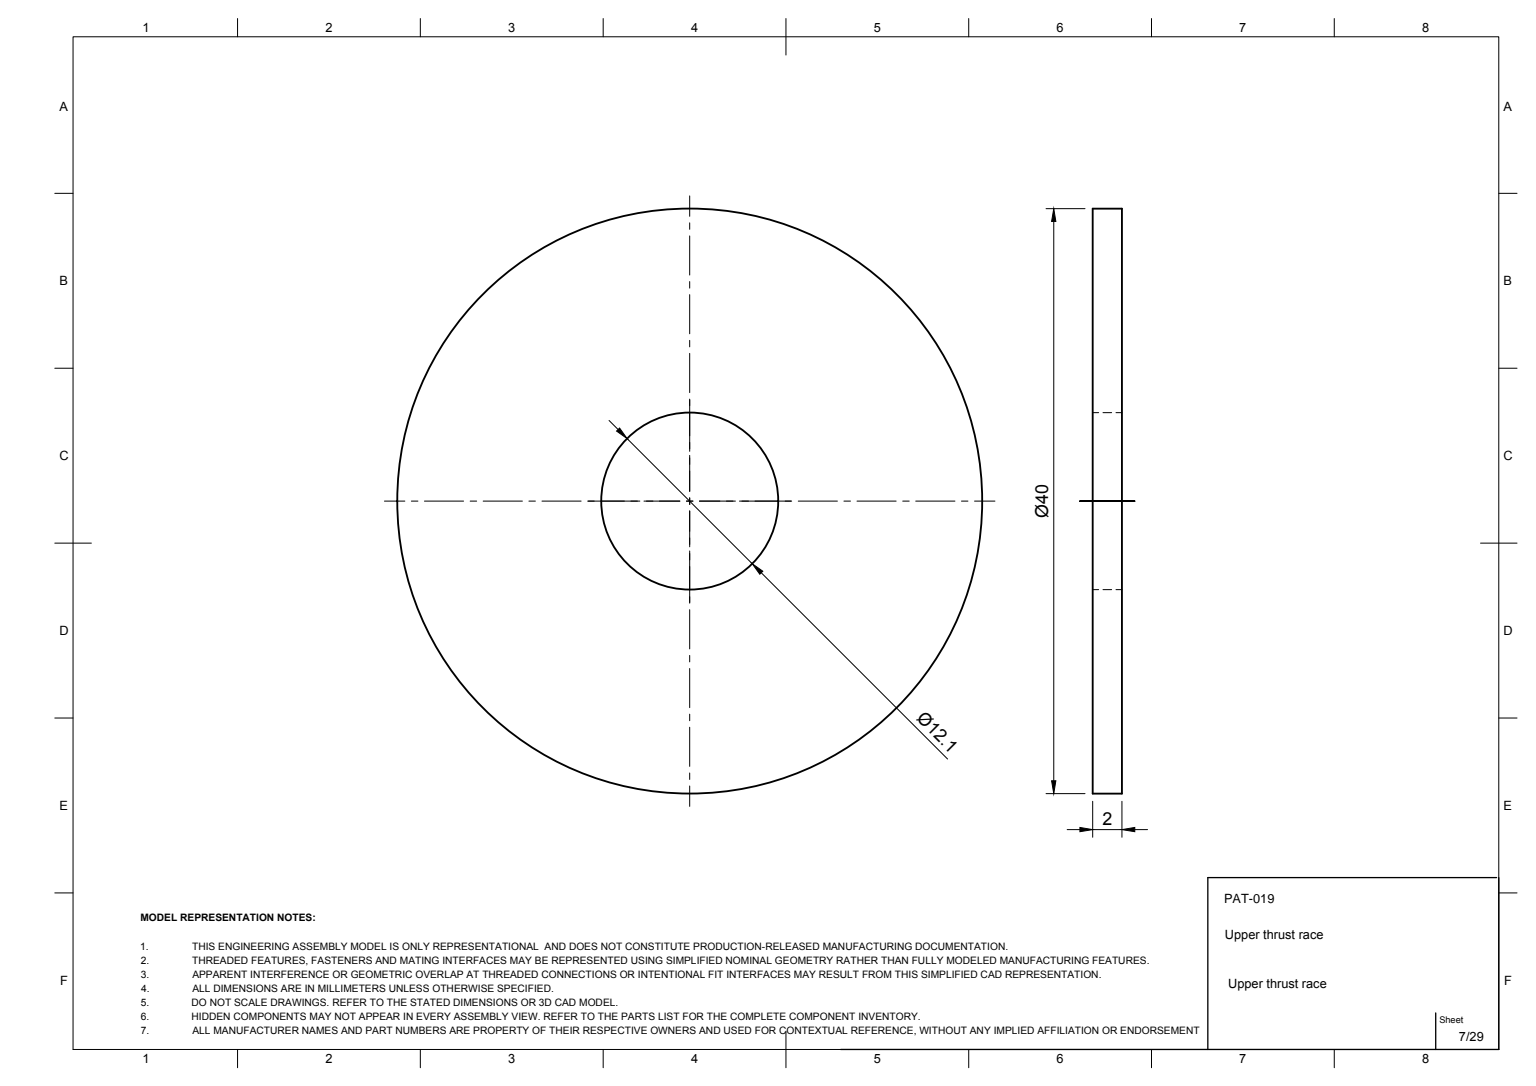
ISO-10303-21;
HEADER;
/* Generated by software containing ST-Developer
 * from STEP Tools, Inc. (www.steptools.com) 
 */

FILE_DESCRIPTION(
/* description */ ('Caster wheel assembly'),
/* implementation_level */ '2;1');

FILE_NAME(
/* name */ 'Upper thrust race.step',
/* time_stamp */ '2026-10-28T03:23:56-07:00',
/* author */ (''),
/* organization */ (''),
/* preprocessor_version */ 'ST-DEVELOPER v20.2',
/* originating_system */ 'Autodesk Translation Framework v15.17.0.0',
/* authorisation */ '');

FILE_SCHEMA (('AUTOMOTIVE_DESIGN { 1 0 10303 214 3 1 1 }'));
ENDSEC;

DATA;
#10=MECHANICAL_DESIGN_GEOMETRIC_PRESENTATION_REPRESENTATION('',(#224),#5385);
#180=SHAPE_REPRESENTATION_RELATIONSHIP('SRR','None',#5475,#202);
#202=ADVANCED_BREP_SHAPE_REPRESENTATION('',(#254),#5362);
#224=STYLED_ITEM('',(#5658),#254);
#254=MANIFOLD_SOLID_BREP('Body1',#2651);
#293=FACE_BOUND('',#622,.T.);
#294=FACE_BOUND('',#624,.T.);
#343=PLANE('',#2968);
#344=PLANE('',#2969);
#439=FACE_OUTER_BOUND('',#619,.T.);
#440=FACE_OUTER_BOUND('',#620,.T.);
#441=FACE_OUTER_BOUND('',#621,.T.);
#442=FACE_OUTER_BOUND('',#623,.T.);
#619=EDGE_LOOP('',(#1854,#1855,#1856,#1857));
#620=EDGE_LOOP('',(#1858,#1859,#1860,#1861));
#621=EDGE_LOOP('',(#1862));
#622=EDGE_LOOP('',(#1863));
#623=EDGE_LOOP('',(#1864));
#624=EDGE_LOOP('',(#1865));
#829=LINE('',#4287,#963);
#830=LINE('',#4293,#964);
#963=VECTOR('',#3406,0.605);
#964=VECTOR('',#3413,2.);
#1093=CIRCLE('',#2963,0.605);
#1094=CIRCLE('',#2964,0.605);
#1095=CIRCLE('',#2966,2.);
#1096=CIRCLE('',#2967,2.);
#1260=VERTEX_POINT('',#4284);
#1261=VERTEX_POINT('',#4286);
#1262=VERTEX_POINT('',#4290);
#1263=VERTEX_POINT('',#4292);
#1495=EDGE_CURVE('',#1260,#1260,#1093,.T.);
#1496=EDGE_CURVE('',#1260,#1261,#829,.T.);
#1497=EDGE_CURVE('',#1261,#1261,#1094,.T.);
#1498=EDGE_CURVE('',#1262,#1262,#1095,.T.);
#1499=EDGE_CURVE('',#1262,#1263,#830,.T.);
#1500=EDGE_CURVE('',#1263,#1263,#1096,.T.);
#1854=ORIENTED_EDGE('',*,*,#1495,.F.);
#1855=ORIENTED_EDGE('',*,*,#1496,.T.);
#1856=ORIENTED_EDGE('',*,*,#1497,.T.);
#1857=ORIENTED_EDGE('',*,*,#1496,.F.);
#1858=ORIENTED_EDGE('',*,*,#1498,.F.);
#1859=ORIENTED_EDGE('',*,*,#1499,.T.);
#1860=ORIENTED_EDGE('',*,*,#1500,.T.);
#1861=ORIENTED_EDGE('',*,*,#1499,.F.);
#1862=ORIENTED_EDGE('',*,*,#1498,.T.);
#1863=ORIENTED_EDGE('',*,*,#1495,.T.);
#1864=ORIENTED_EDGE('',*,*,#1500,.F.);
#1865=ORIENTED_EDGE('',*,*,#1497,.F.);
#2436=CYLINDRICAL_SURFACE('',#2962,0.605);
#2437=CYLINDRICAL_SURFACE('',#2965,2.);
#2499=ADVANCED_FACE('',(#439),#2436,.F.);
#2500=ADVANCED_FACE('',(#440),#2437,.T.);
#2501=ADVANCED_FACE('',(#441,#293),#343,.T.);
#2502=ADVANCED_FACE('',(#442,#294),#344,.F.);
#2651=CLOSED_SHELL('',(#2499,#2500,#2501,#2502));
#2961=AXIS2_PLACEMENT_3D('',#4282,#3400,#3401);
#2962=AXIS2_PLACEMENT_3D('',#4283,#3402,#3403);
#2963=AXIS2_PLACEMENT_3D('',#4285,#3404,#3405);
#2964=AXIS2_PLACEMENT_3D('',#4288,#3407,#3408);
#2965=AXIS2_PLACEMENT_3D('',#4289,#3409,#3410);
#2966=AXIS2_PLACEMENT_3D('',#4291,#3411,#3412);
#2967=AXIS2_PLACEMENT_3D('',#4294,#3414,#3415);
#2968=AXIS2_PLACEMENT_3D('',#4295,#3416,#3417);
#2969=AXIS2_PLACEMENT_3D('',#4296,#3418,#3419);
#3400=DIRECTION('axis',(0.,0.,1.));
#3401=DIRECTION('refdir',(1.,0.,0.));
#3402=DIRECTION('center_axis',(0.,0.,1.));
#3403=DIRECTION('ref_axis',(1.,0.,0.));
#3404=DIRECTION('center_axis',(0.,0.,-1.));
#3405=DIRECTION('ref_axis',(1.,0.,0.));
#3406=DIRECTION('',(0.,0.,-1.));
#3407=DIRECTION('center_axis',(0.,0.,-1.));
#3408=DIRECTION('ref_axis',(1.,0.,0.));
#3409=DIRECTION('center_axis',(0.,0.,1.));
#3410=DIRECTION('ref_axis',(1.,0.,0.));
#3411=DIRECTION('center_axis',(0.,0.,1.));
#3412=DIRECTION('ref_axis',(1.,0.,0.));
#3413=DIRECTION('',(0.,0.,-1.));
#3414=DIRECTION('center_axis',(0.,0.,1.));
#3415=DIRECTION('ref_axis',(1.,0.,0.));
#3416=DIRECTION('center_axis',(0.,0.,1.));
#3417=DIRECTION('ref_axis',(1.,0.,0.));
#3418=DIRECTION('center_axis',(0.,0.,1.));
#3419=DIRECTION('ref_axis',(1.,0.,0.));
#4282=CARTESIAN_POINT('',(0.,0.,0.));
#4283=CARTESIAN_POINT('Origin',(-2.,0.,9.5));
#4284=CARTESIAN_POINT('',(-2.605,-7.40911313484149E-17,9.7));
#4285=CARTESIAN_POINT('Origin',(-2.,0.,9.7));
#4286=CARTESIAN_POINT('',(-2.605,-7.40911313484149E-17,9.5));
#4287=CARTESIAN_POINT('',(-2.605,-7.40911313484149E-17,9.5));
#4288=CARTESIAN_POINT('Origin',(-2.,0.,9.5));
#4289=CARTESIAN_POINT('Origin',(-2.,0.,9.5));
#4290=CARTESIAN_POINT('',(-4.,-2.44929359829471E-16,9.7));
#4291=CARTESIAN_POINT('Origin',(-2.,0.,9.7));
#4292=CARTESIAN_POINT('',(-4.,-2.44929359829471E-16,9.5));
#4293=CARTESIAN_POINT('',(-4.,-2.44929359829471E-16,9.5));
#4294=CARTESIAN_POINT('Origin',(-2.,0.,9.5));
#4295=CARTESIAN_POINT('Origin',(-2.,0.,9.7));
#4296=CARTESIAN_POINT('Origin',(-2.,0.,9.5));
#5334=UNCERTAINTY_MEASURE_WITH_UNIT(LENGTH_MEASURE(0.001),#5386,
'DISTANCE_ACCURACY_VALUE',
'Maximum model space distance between geometric entities at asserted c
onnectivities');
#5357=UNCERTAINTY_MEASURE_WITH_UNIT(LENGTH_MEASURE(0.001),#5386,
'DISTANCE_ACCURACY_VALUE',
'Maximum model space distance between geometric entities at asserted c
onnectivities');
#5362=(
GEOMETRIC_REPRESENTATION_CONTEXT(3)
GLOBAL_UNCERTAINTY_ASSIGNED_CONTEXT((#5334))
GLOBAL_UNIT_ASSIGNED_CONTEXT((#5386,#5388,#5389))
REPRESENTATION_CONTEXT('','3D')
);
#5385=(
GEOMETRIC_REPRESENTATION_CONTEXT(3)
GLOBAL_UNCERTAINTY_ASSIGNED_CONTEXT((#5357))
GLOBAL_UNIT_ASSIGNED_CONTEXT((#5386,#5388,#5389))
REPRESENTATION_CONTEXT('','3D')
);
#5386=(
LENGTH_UNIT()
NAMED_UNIT(*)
SI_UNIT(.CENTI.,.METRE.)
);
#5388=(
NAMED_UNIT(*)
PLANE_ANGLE_UNIT()
SI_UNIT($,.RADIAN.)
);
#5389=(
NAMED_UNIT(*)
SI_UNIT($,.STERADIAN.)
SOLID_ANGLE_UNIT()
);
#5394=SHAPE_DEFINITION_REPRESENTATION(#5421,#5475);
#5421=PRODUCT_DEFINITION_SHAPE('',$,#5503);
#5475=SHAPE_REPRESENTATION('',(#2961),#5362);
#5498=PRODUCT_DEFINITION_CONTEXT('part definition',#5581,'design');
#5503=PRODUCT_DEFINITION('Upper thrust race','Upper thrust race',#5530,
#5498);
#5530=PRODUCT_DEFINITION_FORMATION('',$,#5587);
#5581=APPLICATION_CONTEXT(
'Core Data for Automotive Mechanical Design Process');
#5582=PRODUCT_CONTEXT('part definition',#5581,'mechanical');
#5587=PRODUCT('Upper thrust race','Upper thrust race',
'Upper thrust race',(#5582));
#5652=COLOUR_RGB('Light Blue',0.38,0.62,0.78);
#5653=FILL_AREA_STYLE_COLOUR('',#5652);
#5654=FILL_AREA_STYLE('',(#5653));
#5655=SURFACE_STYLE_FILL_AREA(#5654);
#5656=SURFACE_SIDE_STYLE('',(#5655));
#5657=SURFACE_STYLE_USAGE(.BOTH.,#5656);
#5658=PRESENTATION_STYLE_ASSIGNMENT((#5657));
ENDSEC;
END-ISO-10303-21;
